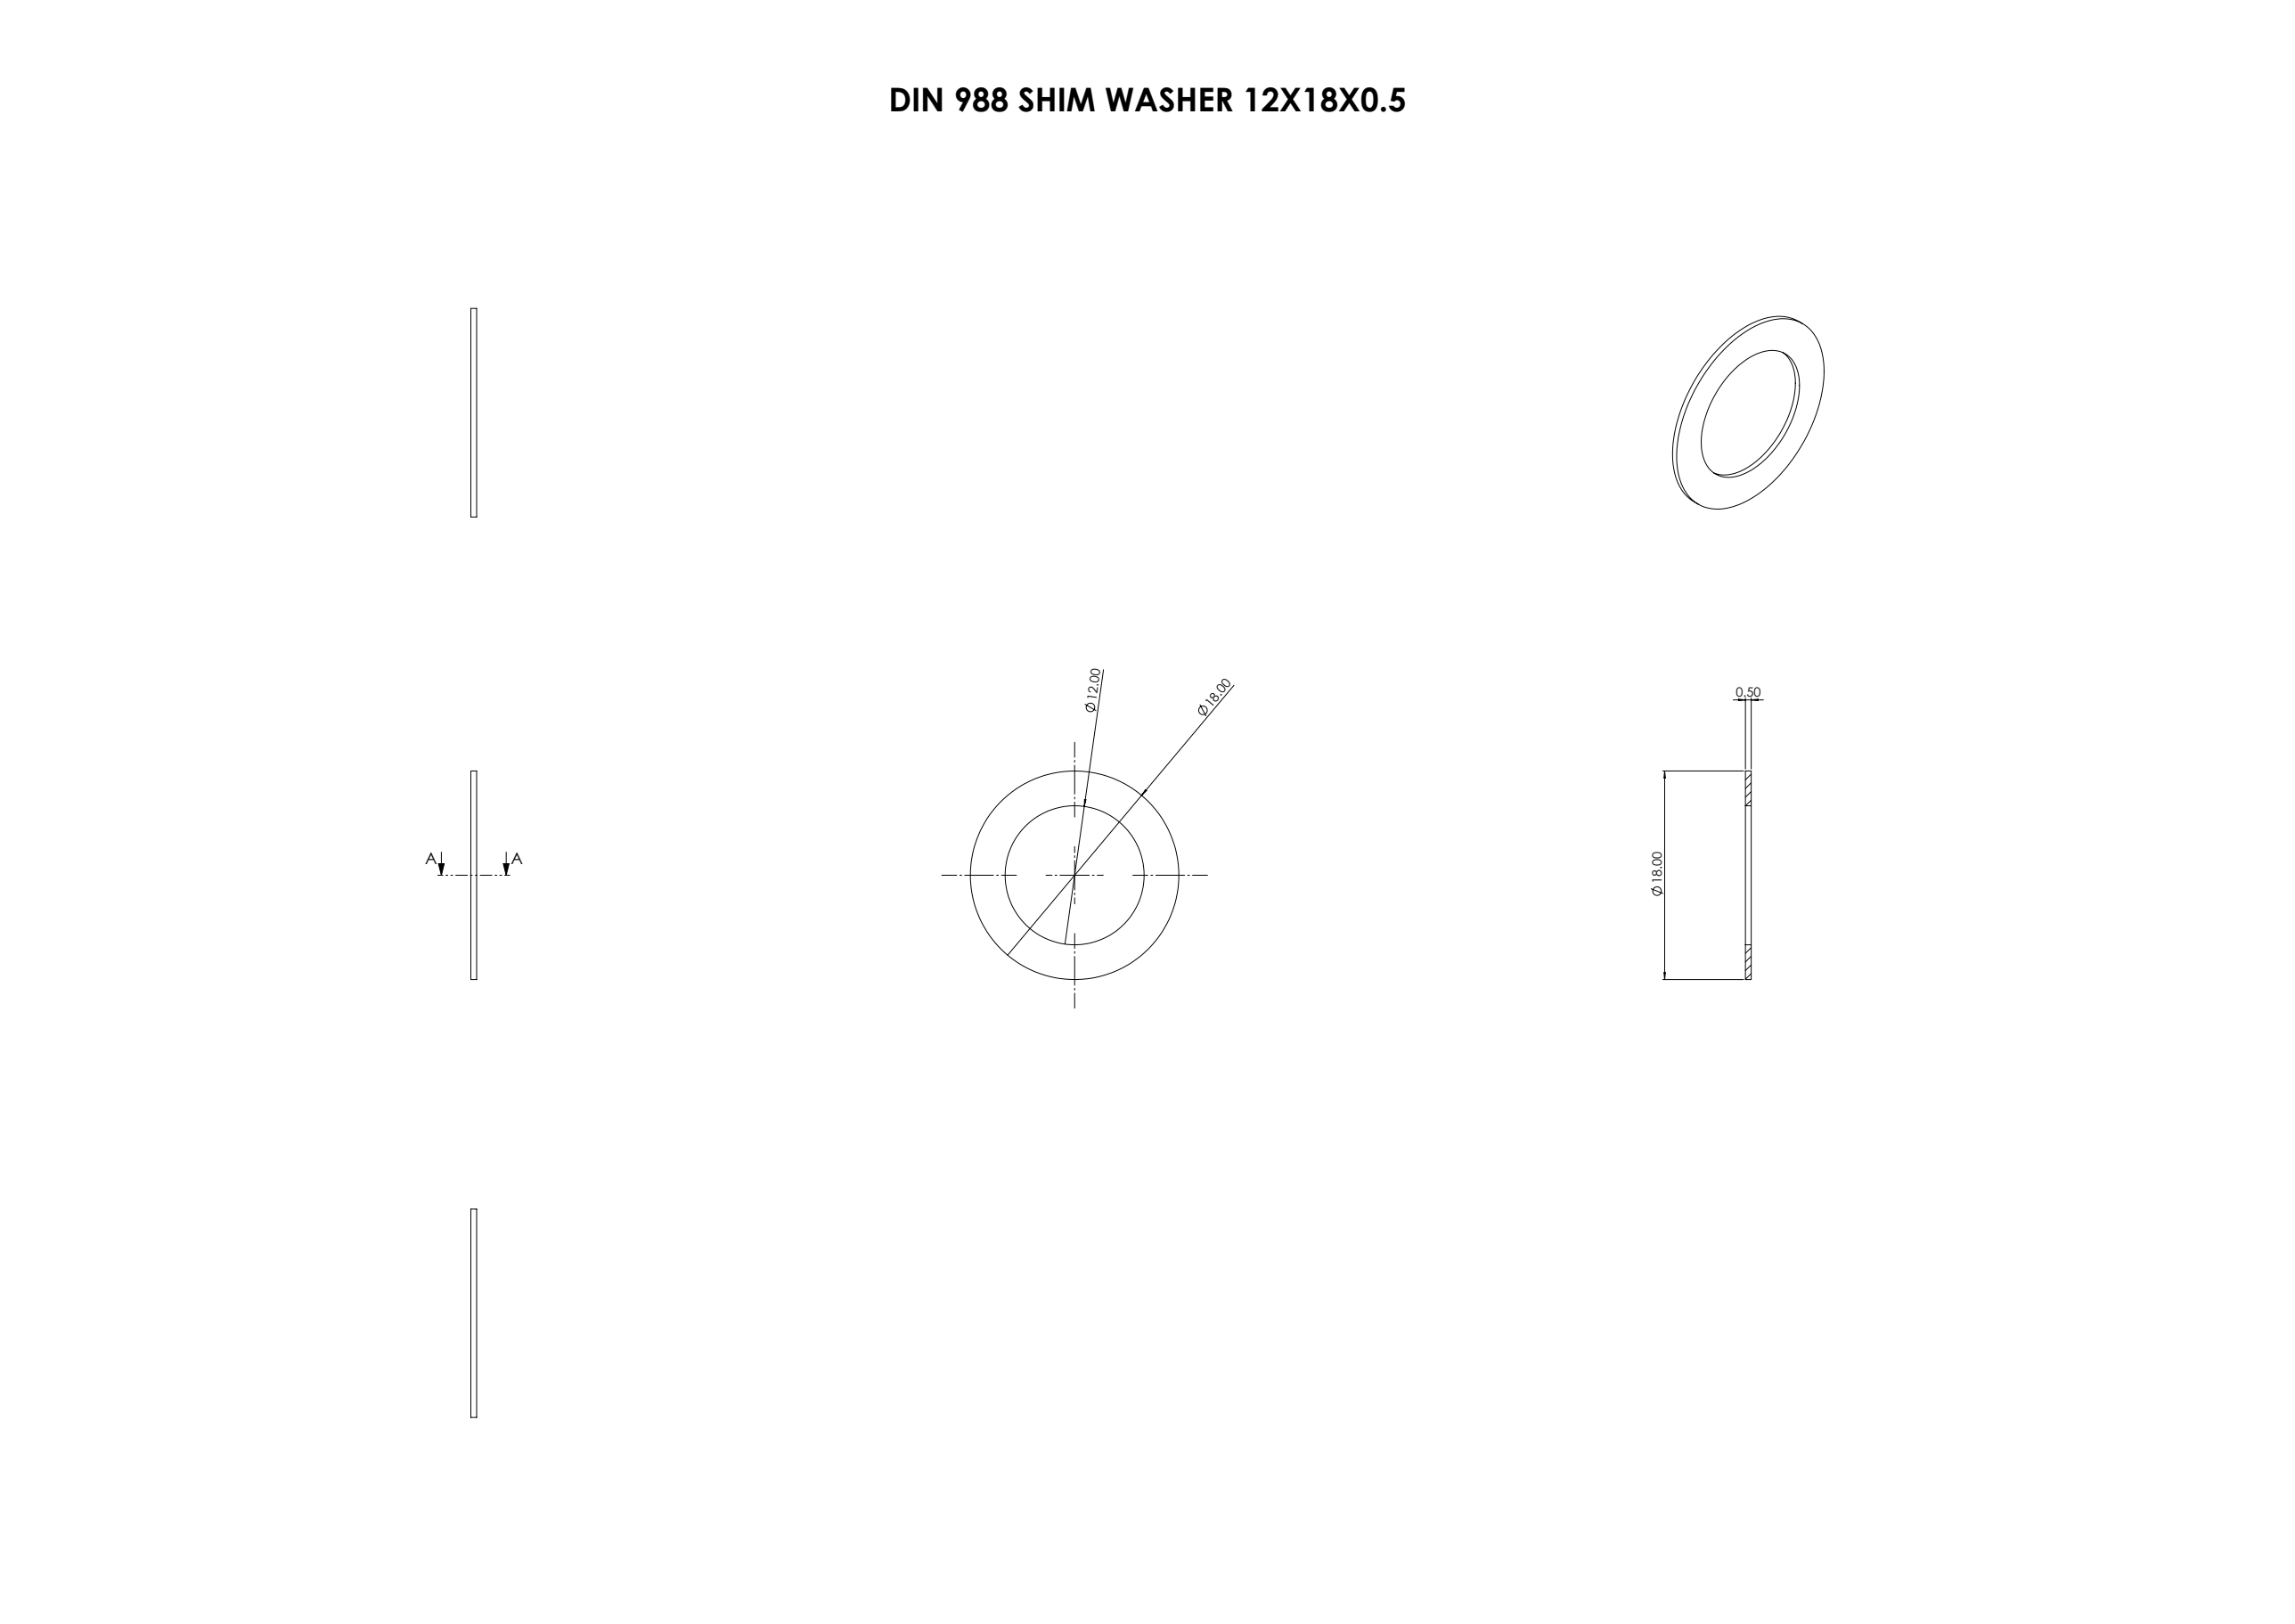
ISO-10303-21;
HEADER;
/* Generated by software containing ST-Developer
 * from STEP Tools, Inc. (www.steptools.com) 
 */

FILE_DESCRIPTION(
/* description */ (''),
/* implementation_level */ '2;1');

FILE_NAME(
/* name */ '08_DIN_988_Shim_Washer_12x18x0.5.step',
/* time_stamp */ '2026-10-11T09:12:28-07:00',
/* author */ (''),
/* organization */ (''),
/* preprocessor_version */ 'ST-DEVELOPER v20.2',
/* originating_system */ 'Autodesk Translation Framework v15.15.0.0',
/* authorisation */ '');

FILE_SCHEMA (('AUTOMOTIVE_DESIGN { 1 0 10303 214 3 1 1 }'));
ENDSEC;

DATA;
#10=MECHANICAL_DESIGN_GEOMETRIC_PRESENTATION_REPRESENTATION('',(#654),#23254);
#634=SHAPE_REPRESENTATION_RELATIONSHIP('SRR','None',#23307,#644);
#644=ADVANCED_BREP_SHAPE_REPRESENTATION('',(#664),#23251);
#654=STYLED_ITEM('',(#23469),#664);
#664=MANIFOLD_SOLID_BREP('Body1',#7032);
#844=FACE_BOUND('',#1792,.T.);
#845=FACE_BOUND('',#1795,.T.);
#958=PLANE('',#7750);
#959=PLANE('',#7754);
#1331=FACE_OUTER_BOUND('',#1790,.T.);
#1332=FACE_OUTER_BOUND('',#1791,.T.);
#1333=FACE_OUTER_BOUND('',#1793,.T.);
#1334=FACE_OUTER_BOUND('',#1794,.T.);
#1790=EDGE_LOOP('',(#6361,#6362,#6363,#6364));
#1791=EDGE_LOOP('',(#6365));
#1792=EDGE_LOOP('',(#6366));
#1793=EDGE_LOOP('',(#6367,#6368,#6369,#6370));
#1794=EDGE_LOOP('',(#6371));
#1795=EDGE_LOOP('',(#6372));
#2046=LINE('',#22077,#2305);
#2047=LINE('',#22084,#2306);
#2305=VECTOR('',#9242,9.);
#2306=VECTOR('',#9251,6.);
#2679=CIRCLE('',#7748,9.);
#2680=CIRCLE('',#7749,9.);
#2681=CIRCLE('',#7751,6.);
#2682=CIRCLE('',#7753,6.);
#3337=VERTEX_POINT('',#22074);
#3338=VERTEX_POINT('',#22076);
#3339=VERTEX_POINT('',#22080);
#3340=VERTEX_POINT('',#22083);
#4356=EDGE_CURVE('',#3337,#3337,#2679,.T.);
#4357=EDGE_CURVE('',#3337,#3338,#2046,.T.);
#4358=EDGE_CURVE('',#3338,#3338,#2680,.T.);
#4359=EDGE_CURVE('',#3339,#3339,#2681,.T.);
#4360=EDGE_CURVE('',#3339,#3340,#2047,.T.);
#4361=EDGE_CURVE('',#3340,#3340,#2682,.T.);
#6361=ORIENTED_EDGE('',*,*,#4356,.F.);
#6362=ORIENTED_EDGE('',*,*,#4357,.T.);
#6363=ORIENTED_EDGE('',*,*,#4358,.T.);
#6364=ORIENTED_EDGE('',*,*,#4357,.F.);
#6365=ORIENTED_EDGE('',*,*,#4356,.T.);
#6366=ORIENTED_EDGE('',*,*,#4359,.F.);
#6367=ORIENTED_EDGE('',*,*,#4359,.T.);
#6368=ORIENTED_EDGE('',*,*,#4360,.T.);
#6369=ORIENTED_EDGE('',*,*,#4361,.F.);
#6370=ORIENTED_EDGE('',*,*,#4360,.F.);
#6371=ORIENTED_EDGE('',*,*,#4358,.F.);
#6372=ORIENTED_EDGE('',*,*,#4361,.T.);
#6613=CYLINDRICAL_SURFACE('',#7747,9.);
#6614=CYLINDRICAL_SURFACE('',#7752,6.);
#6982=ADVANCED_FACE('',(#1331),#6613,.T.);
#6983=ADVANCED_FACE('',(#1332,#844),#958,.T.);
#6984=ADVANCED_FACE('',(#1333),#6614,.F.);
#6985=ADVANCED_FACE('',(#1334,#845),#959,.T.);
#7032=CLOSED_SHELL('',(#6982,#6983,#6984,#6985));
#7746=AXIS2_PLACEMENT_3D('',#22072,#9236,#9237);
#7747=AXIS2_PLACEMENT_3D('',#22073,#9238,#9239);
#7748=AXIS2_PLACEMENT_3D('',#22075,#9240,#9241);
#7749=AXIS2_PLACEMENT_3D('',#22078,#9243,#9244);
#7750=AXIS2_PLACEMENT_3D('',#22079,#9245,#9246);
#7751=AXIS2_PLACEMENT_3D('',#22081,#9247,#9248);
#7752=AXIS2_PLACEMENT_3D('',#22082,#9249,#9250);
#7753=AXIS2_PLACEMENT_3D('',#22085,#9252,#9253);
#7754=AXIS2_PLACEMENT_3D('',#22086,#9254,#9255);
#9236=DIRECTION('axis',(0.,0.,1.));
#9237=DIRECTION('refdir',(1.,0.,0.));
#9238=DIRECTION('center_axis',(1.,0.,0.));
#9239=DIRECTION('ref_axis',(0.,1.,0.));
#9240=DIRECTION('center_axis',(1.,0.,0.));
#9241=DIRECTION('ref_axis',(0.,0.,-1.));
#9242=DIRECTION('',(-1.,0.,0.));
#9243=DIRECTION('center_axis',(1.,0.,0.));
#9244=DIRECTION('ref_axis',(0.,0.,-1.));
#9245=DIRECTION('center_axis',(1.,0.,0.));
#9246=DIRECTION('ref_axis',(0.,0.,-1.));
#9247=DIRECTION('center_axis',(1.,0.,0.));
#9248=DIRECTION('ref_axis',(0.,0.,-1.));
#9249=DIRECTION('center_axis',(1.,0.,0.));
#9250=DIRECTION('ref_axis',(0.,1.,0.));
#9251=DIRECTION('',(-1.,0.,0.));
#9252=DIRECTION('center_axis',(1.,0.,0.));
#9253=DIRECTION('ref_axis',(0.,0.,-1.));
#9254=DIRECTION('center_axis',(-1.,0.,0.));
#9255=DIRECTION('ref_axis',(0.,0.,1.));
#22072=CARTESIAN_POINT('',(0.,0.,0.));
#22073=CARTESIAN_POINT('Origin',(0.25,0.,0.));
#22074=CARTESIAN_POINT('',(0.5,-9.,-1.10218211923262E-15));
#22075=CARTESIAN_POINT('Origin',(0.5,0.,0.));
#22076=CARTESIAN_POINT('',(0.,-9.,-1.10218211923262E-15));
#22077=CARTESIAN_POINT('',(0.25,-9.,-1.10218211923262E-15));
#22078=CARTESIAN_POINT('Origin',(0.,0.,0.));
#22079=CARTESIAN_POINT('Origin',(0.5,6.,0.));
#22080=CARTESIAN_POINT('',(0.5,-6.,-7.34788079488412E-16));
#22081=CARTESIAN_POINT('Origin',(0.5,0.,0.));
#22082=CARTESIAN_POINT('Origin',(0.25,0.,0.));
#22083=CARTESIAN_POINT('',(0.,-6.,-7.34788079488412E-16));
#22084=CARTESIAN_POINT('',(0.25,-6.,-7.34788079488412E-16));
#22085=CARTESIAN_POINT('Origin',(0.,0.,0.));
#22086=CARTESIAN_POINT('Origin',(0.,9.,0.));
#23239=UNCERTAINTY_MEASURE_WITH_UNIT(LENGTH_MEASURE(0.01),#23255,
'DISTANCE_ACCURACY_VALUE',
'Maximum model space distance between geometric entities at asserted c
onnectivities');
#23242=UNCERTAINTY_MEASURE_WITH_UNIT(LENGTH_MEASURE(0.01),#23255,
'DISTANCE_ACCURACY_VALUE',
'Maximum model space distance between geometric entities at asserted c
onnectivities');
#23251=(
GEOMETRIC_REPRESENTATION_CONTEXT(3)
GLOBAL_UNCERTAINTY_ASSIGNED_CONTEXT((#23239))
GLOBAL_UNIT_ASSIGNED_CONTEXT((#23255,#23257,#23258))
REPRESENTATION_CONTEXT('','3D')
);
#23254=(
GEOMETRIC_REPRESENTATION_CONTEXT(3)
GLOBAL_UNCERTAINTY_ASSIGNED_CONTEXT((#23242))
GLOBAL_UNIT_ASSIGNED_CONTEXT((#23255,#23257,#23258))
REPRESENTATION_CONTEXT('','3D')
);
#23255=(
LENGTH_UNIT()
NAMED_UNIT(*)
SI_UNIT(.MILLI.,.METRE.)
);
#23257=(
NAMED_UNIT(*)
PLANE_ANGLE_UNIT()
SI_UNIT($,.RADIAN.)
);
#23258=(
NAMED_UNIT(*)
SI_UNIT($,.STERADIAN.)
SOLID_ANGLE_UNIT()
);
#23267=SHAPE_DEFINITION_REPRESENTATION(#23278,#23307);
#23278=PRODUCT_DEFINITION_SHAPE('',$,#23319);
#23307=SHAPE_REPRESENTATION('',(#7746),#23251);
#23310=PRODUCT_DEFINITION_CONTEXT('part definition',#23345,'design');
#23319=PRODUCT_DEFINITION('2026-10-11-09-11-54-876',
'08_DIN_988_Shim_Washer_12x18x0.5',#23330,#23310);
#23330=PRODUCT_DEFINITION_FORMATION('',$,#23355);
#23345=APPLICATION_CONTEXT(
'Core Data for Automotive Mechanical Design Process');
#23346=PRODUCT_CONTEXT('part definition',#23345,'mechanical');
#23355=PRODUCT('2026-10-11-09-11-54-876',
'08_DIN_988_Shim_Washer_12x18x0.5',$,(#23346));
#23463=COLOUR_RGB('Black',0.12,0.14,0.17);
#23464=FILL_AREA_STYLE_COLOUR('',#23463);
#23465=FILL_AREA_STYLE('',(#23464));
#23466=SURFACE_STYLE_FILL_AREA(#23465);
#23467=SURFACE_SIDE_STYLE('',(#23466));
#23468=SURFACE_STYLE_USAGE(.BOTH.,#23467);
#23469=PRESENTATION_STYLE_ASSIGNMENT((#23468));
ENDSEC;
END-ISO-10303-21;
